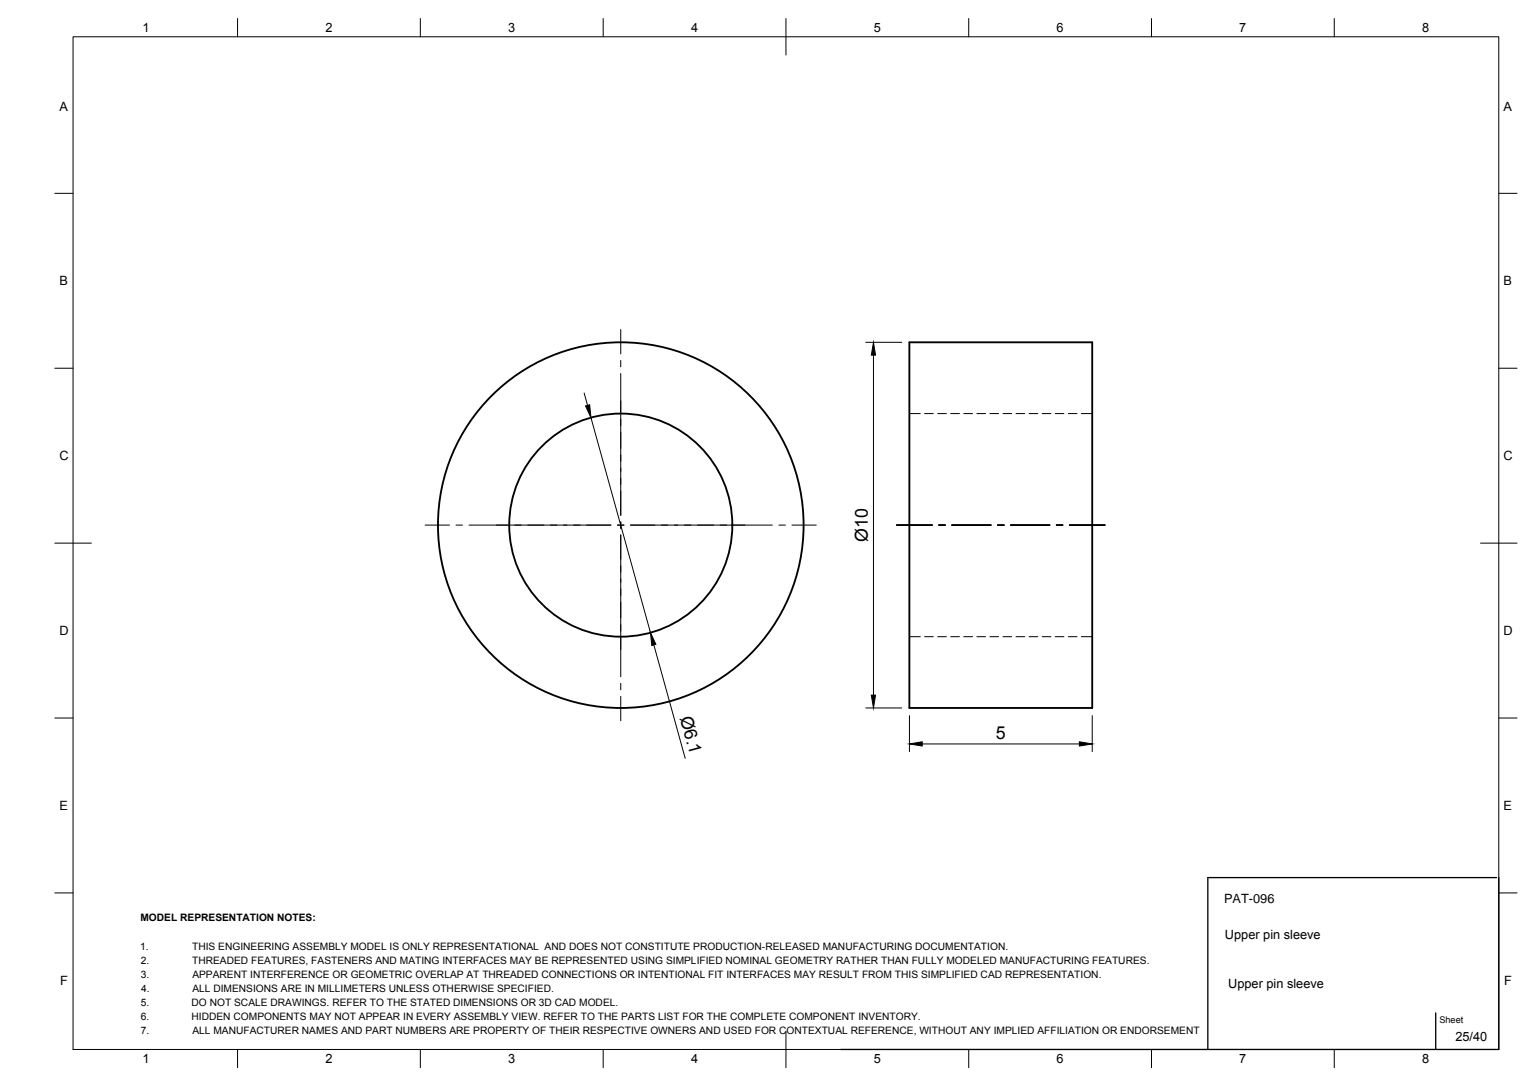
ISO-10303-21;
HEADER;
/* Generated by software containing ST-Developer
 * from STEP Tools, Inc. (www.steptools.com) 
 */

FILE_DESCRIPTION(
/* description */ ('PAT-096'),
/* implementation_level */ '2;1');

FILE_NAME(
/* name */ 'Upper pin sleeve.step',
/* time_stamp */ '2026-10-29T17:03:14-07:00',
/* author */ (''),
/* organization */ (''),
/* preprocessor_version */ 'ST-DEVELOPER v20.2',
/* originating_system */ 'Autodesk Translation Framework v15.17.0.0',
/* authorisation */ '');

FILE_SCHEMA (('AUTOMOTIVE_DESIGN { 1 0 10303 214 3 1 1 }'));
ENDSEC;

DATA;
#10=MECHANICAL_DESIGN_GEOMETRIC_PRESENTATION_REPRESENTATION('',(#434),#10650);
#364=SHAPE_REPRESENTATION_RELATIONSHIP('SRR','None',#10829,#395);
#395=ADVANCED_BREP_SHAPE_REPRESENTATION('',(#471),#10647);
#434=STYLED_ITEM('',(#11064),#471);
#471=MANIFOLD_SOLID_BREP('Body1',#5569);
#607=FACE_BOUND('',#1575,.T.);
#608=FACE_BOUND('',#1577,.T.);
#775=PLANE('',#6583);
#776=PLANE('',#6584);
#1102=FACE_OUTER_BOUND('',#1572,.T.);
#1103=FACE_OUTER_BOUND('',#1573,.T.);
#1104=FACE_OUTER_BOUND('',#1574,.T.);
#1105=FACE_OUTER_BOUND('',#1576,.T.);
#1572=EDGE_LOOP('',(#4989,#4990,#4991,#4992));
#1573=EDGE_LOOP('',(#4993,#4994,#4995,#4996));
#1574=EDGE_LOOP('',(#4997));
#1575=EDGE_LOOP('',(#4998));
#1576=EDGE_LOOP('',(#4999));
#1577=EDGE_LOOP('',(#5000));
#1903=LINE('',#10429,#2232);
#1904=LINE('',#10435,#2233);
#2232=VECTOR('',#8301,0.305);
#2233=VECTOR('',#8308,0.5);
#2563=CIRCLE('',#6578,0.305);
#2564=CIRCLE('',#6579,0.305);
#2565=CIRCLE('',#6581,0.5);
#2566=CIRCLE('',#6582,0.5);
#3009=VERTEX_POINT('',#10426);
#3010=VERTEX_POINT('',#10428);
#3011=VERTEX_POINT('',#10432);
#3012=VERTEX_POINT('',#10434);
#3673=EDGE_CURVE('',#3009,#3009,#2563,.T.);
#3674=EDGE_CURVE('',#3009,#3010,#1903,.T.);
#3675=EDGE_CURVE('',#3010,#3010,#2564,.T.);
#3676=EDGE_CURVE('',#3011,#3011,#2565,.T.);
#3677=EDGE_CURVE('',#3011,#3012,#1904,.T.);
#3678=EDGE_CURVE('',#3012,#3012,#2566,.T.);
#4989=ORIENTED_EDGE('',*,*,#3673,.F.);
#4990=ORIENTED_EDGE('',*,*,#3674,.T.);
#4991=ORIENTED_EDGE('',*,*,#3675,.T.);
#4992=ORIENTED_EDGE('',*,*,#3674,.F.);
#4993=ORIENTED_EDGE('',*,*,#3676,.F.);
#4994=ORIENTED_EDGE('',*,*,#3677,.T.);
#4995=ORIENTED_EDGE('',*,*,#3678,.T.);
#4996=ORIENTED_EDGE('',*,*,#3677,.F.);
#4997=ORIENTED_EDGE('',*,*,#3676,.T.);
#4998=ORIENTED_EDGE('',*,*,#3673,.T.);
#4999=ORIENTED_EDGE('',*,*,#3678,.F.);
#5000=ORIENTED_EDGE('',*,*,#3675,.F.);
#5189=CYLINDRICAL_SURFACE('',#6577,0.305);
#5190=CYLINDRICAL_SURFACE('',#6580,0.5);
#5507=ADVANCED_FACE('',(#1102),#5189,.F.);
#5508=ADVANCED_FACE('',(#1103),#5190,.T.);
#5509=ADVANCED_FACE('',(#1104,#607),#775,.T.);
#5510=ADVANCED_FACE('',(#1105,#608),#776,.F.);
#5569=CLOSED_SHELL('',(#5507,#5508,#5509,#5510));
#6576=AXIS2_PLACEMENT_3D('',#10424,#8295,#8296);
#6577=AXIS2_PLACEMENT_3D('',#10425,#8297,#8298);
#6578=AXIS2_PLACEMENT_3D('',#10427,#8299,#8300);
#6579=AXIS2_PLACEMENT_3D('',#10430,#8302,#8303);
#6580=AXIS2_PLACEMENT_3D('',#10431,#8304,#8305);
#6581=AXIS2_PLACEMENT_3D('',#10433,#8306,#8307);
#6582=AXIS2_PLACEMENT_3D('',#10436,#8309,#8310);
#6583=AXIS2_PLACEMENT_3D('',#10437,#8311,#8312);
#6584=AXIS2_PLACEMENT_3D('',#10438,#8313,#8314);
#8295=DIRECTION('axis',(0.,0.,1.));
#8296=DIRECTION('refdir',(1.,0.,0.));
#8297=DIRECTION('center_axis',(0.,0.,1.));
#8298=DIRECTION('ref_axis',(1.,0.,0.));
#8299=DIRECTION('center_axis',(0.,0.,-1.));
#8300=DIRECTION('ref_axis',(1.,0.,0.));
#8301=DIRECTION('',(0.,0.,-1.));
#8302=DIRECTION('center_axis',(0.,0.,-1.));
#8303=DIRECTION('ref_axis',(1.,0.,0.));
#8304=DIRECTION('center_axis',(0.,0.,1.));
#8305=DIRECTION('ref_axis',(1.,0.,0.));
#8306=DIRECTION('center_axis',(0.,0.,1.));
#8307=DIRECTION('ref_axis',(1.,0.,0.));
#8308=DIRECTION('',(0.,0.,-1.));
#8309=DIRECTION('center_axis',(0.,0.,1.));
#8310=DIRECTION('ref_axis',(1.,0.,0.));
#8311=DIRECTION('center_axis',(0.,0.,1.));
#8312=DIRECTION('ref_axis',(1.,0.,0.));
#8313=DIRECTION('center_axis',(0.,0.,1.));
#8314=DIRECTION('ref_axis',(1.,0.,0.));
#10424=CARTESIAN_POINT('',(0.,0.,0.));
#10425=CARTESIAN_POINT('Origin',(0.,2.,9.6));
#10426=CARTESIAN_POINT('',(-0.305,2.,10.1));
#10427=CARTESIAN_POINT('Origin',(0.,2.,10.1));
#10428=CARTESIAN_POINT('',(-0.305,2.,9.6));
#10429=CARTESIAN_POINT('',(-0.305,2.,9.6));
#10430=CARTESIAN_POINT('Origin',(0.,2.,9.6));
#10431=CARTESIAN_POINT('Origin',(0.,2.,9.6));
#10432=CARTESIAN_POINT('',(-0.5,2.,10.1));
#10433=CARTESIAN_POINT('Origin',(0.,2.,10.1));
#10434=CARTESIAN_POINT('',(-0.5,2.,9.6));
#10435=CARTESIAN_POINT('',(-0.5,2.,9.6));
#10436=CARTESIAN_POINT('Origin',(0.,2.,9.6));
#10437=CARTESIAN_POINT('Origin',(0.,2.,10.1));
#10438=CARTESIAN_POINT('Origin',(0.,2.,9.6));
#10608=UNCERTAINTY_MEASURE_WITH_UNIT(LENGTH_MEASURE(0.001),#10651,
'DISTANCE_ACCURACY_VALUE',
'Maximum model space distance between geometric entities at asserted c
onnectivities');
#10611=UNCERTAINTY_MEASURE_WITH_UNIT(LENGTH_MEASURE(0.001),#10651,
'DISTANCE_ACCURACY_VALUE',
'Maximum model space distance between geometric entities at asserted c
onnectivities');
#10647=(
GEOMETRIC_REPRESENTATION_CONTEXT(3)
GLOBAL_UNCERTAINTY_ASSIGNED_CONTEXT((#10608))
GLOBAL_UNIT_ASSIGNED_CONTEXT((#10651,#10653,#10654))
REPRESENTATION_CONTEXT('','3D')
);
#10650=(
GEOMETRIC_REPRESENTATION_CONTEXT(3)
GLOBAL_UNCERTAINTY_ASSIGNED_CONTEXT((#10611))
GLOBAL_UNIT_ASSIGNED_CONTEXT((#10651,#10653,#10654))
REPRESENTATION_CONTEXT('','3D')
);
#10651=(
LENGTH_UNIT()
NAMED_UNIT(*)
SI_UNIT(.CENTI.,.METRE.)
);
#10653=(
NAMED_UNIT(*)
PLANE_ANGLE_UNIT()
SI_UNIT($,.RADIAN.)
);
#10654=(
NAMED_UNIT(*)
SI_UNIT($,.STERADIAN.)
SOLID_ANGLE_UNIT()
);
#10690=SHAPE_DEFINITION_REPRESENTATION(#10738,#10829);
#10738=PRODUCT_DEFINITION_SHAPE('',$,#10868);
#10829=SHAPE_REPRESENTATION('',(#6576),#10647);
#10832=PRODUCT_DEFINITION_CONTEXT('part definition',#10948,'design');
#10868=PRODUCT_DEFINITION('Upper pin sleeve','Upper pin sleeve',#10906,
#10832);
#10906=PRODUCT_DEFINITION_FORMATION('',$,#10985);
#10948=APPLICATION_CONTEXT(
'Core Data for Automotive Mechanical Design Process');
#10949=PRODUCT_CONTEXT('part definition',#10948,'mechanical');
#10985=PRODUCT('Upper pin sleeve','Upper pin sleeve','Upper pin sleeve',
(#10949));
#11058=COLOUR_RGB('Grey',0.48,0.52,0.57);
#11059=FILL_AREA_STYLE_COLOUR('',#11058);
#11060=FILL_AREA_STYLE('',(#11059));
#11061=SURFACE_STYLE_FILL_AREA(#11060);
#11062=SURFACE_SIDE_STYLE('',(#11061));
#11063=SURFACE_STYLE_USAGE(.BOTH.,#11062);
#11064=PRESENTATION_STYLE_ASSIGNMENT((#11063));
ENDSEC;
END-ISO-10303-21;
